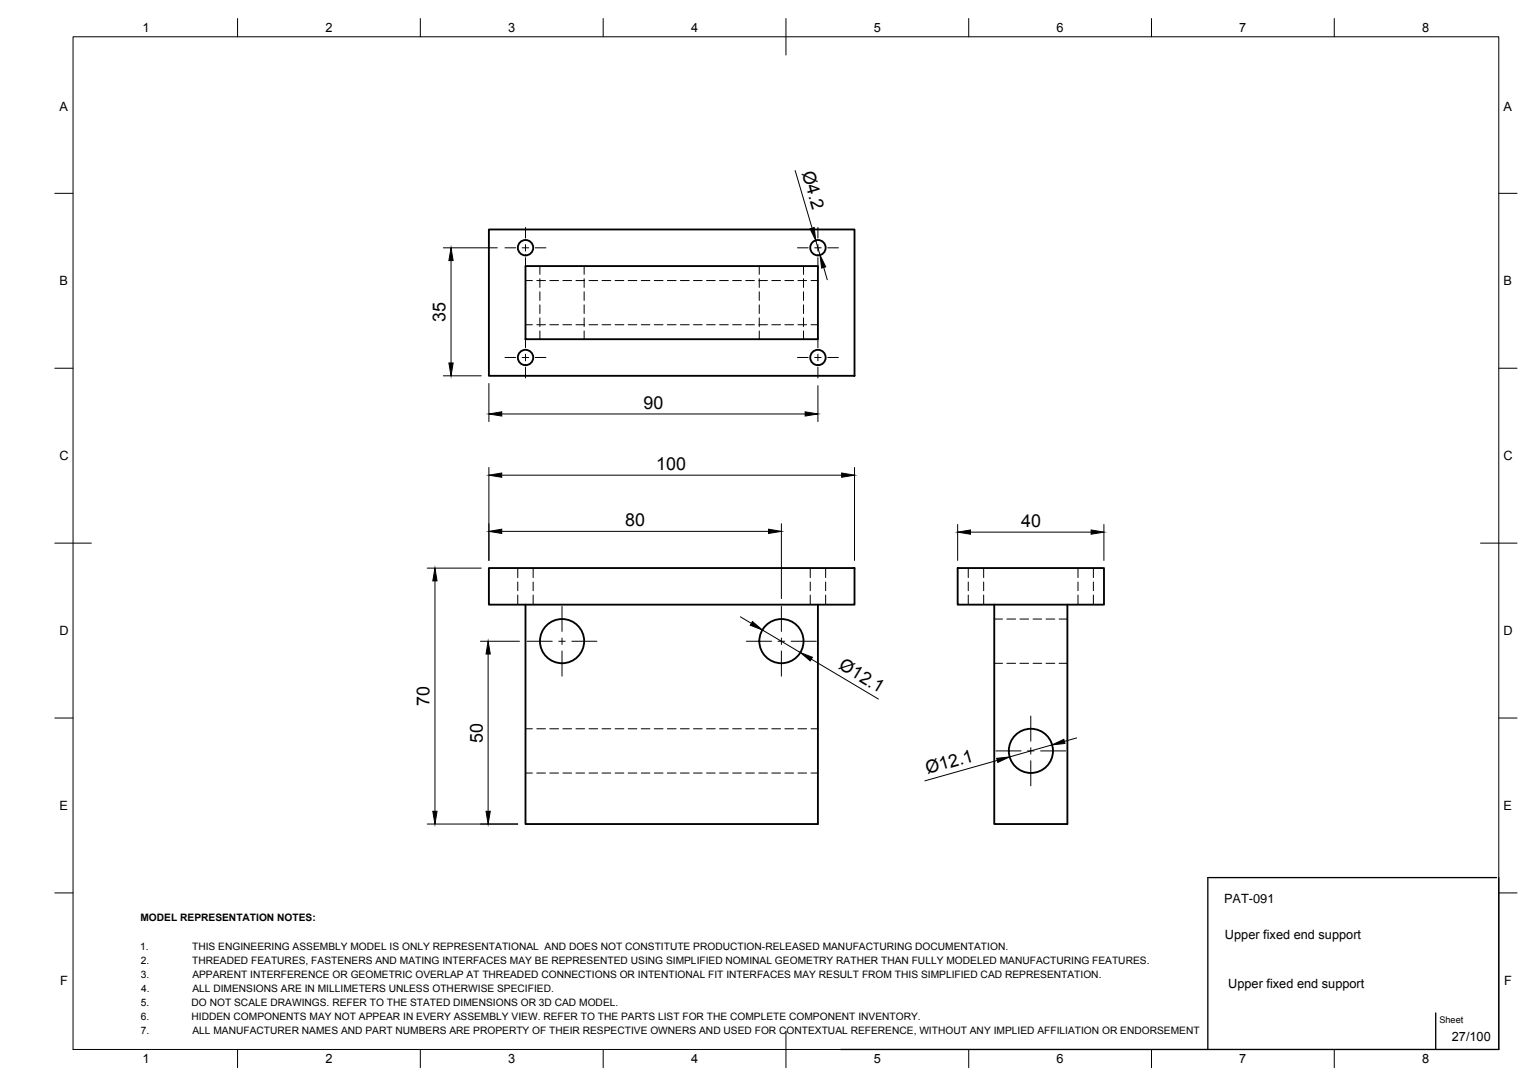
ISO-10303-21;
HEADER;
/* Generated by software containing ST-Developer
 * from STEP Tools, Inc. (www.steptools.com) 
 */

FILE_DESCRIPTION(
/* description */ ('PAT-091'),
/* implementation_level */ '2;1');

FILE_NAME(
/* name */ 'Upper fixed end support.step',
/* time_stamp */ '2026-10-27T15:34:44-07:00',
/* author */ (''),
/* organization */ (''),
/* preprocessor_version */ 'ST-DEVELOPER v20.2',
/* originating_system */ 'Autodesk Translation Framework v15.17.0.0',
/* authorisation */ '');

FILE_SCHEMA (('AUTOMOTIVE_DESIGN { 1 0 10303 214 3 1 1 }'));
ENDSEC;

DATA;
#10=MECHANICAL_DESIGN_GEOMETRIC_PRESENTATION_REPRESENTATION('',(#990),#25100);
#770=SHAPE_REPRESENTATION_RELATIONSHIP('SRR','None',#25532,#880);
#880=ADVANCED_BREP_SHAPE_REPRESENTATION('',(#1113),#25002);
#990=STYLED_ITEM('',(#26184),#1113);
#1113=MANIFOLD_SOLID_BREP('Body1',#13268);
#1350=FACE_BOUND('',#3193,.T.);
#1351=FACE_BOUND('',#3194,.T.);
#1352=FACE_BOUND('',#3195,.T.);
#1353=FACE_BOUND('',#3196,.T.);
#1354=FACE_BOUND('',#3197,.T.);
#1355=FACE_BOUND('',#3203,.T.);
#1356=FACE_BOUND('',#3205,.T.);
#1357=FACE_BOUND('',#3206,.T.);
#1358=FACE_BOUND('',#3211,.T.);
#1359=FACE_BOUND('',#3213,.T.);
#1360=FACE_BOUND('',#3214,.T.);
#1361=FACE_BOUND('',#3216,.T.);
#1362=FACE_BOUND('',#3217,.T.);
#1363=FACE_BOUND('',#3218,.T.);
#1364=FACE_BOUND('',#3219,.T.);
#1725=PLANE('',#14963);
#1726=PLANE('',#14964);
#1727=PLANE('',#14965);
#1728=PLANE('',#14966);
#1729=PLANE('',#14967);
#1730=PLANE('',#14968);
#1731=PLANE('',#14970);
#1732=PLANE('',#14979);
#1733=PLANE('',#14980);
#1734=PLANE('',#14981);
#1735=PLANE('',#14982);
#2235=FACE_OUTER_BOUND('',#3188,.T.);
#2236=FACE_OUTER_BOUND('',#3189,.T.);
#2237=FACE_OUTER_BOUND('',#3190,.T.);
#2238=FACE_OUTER_BOUND('',#3191,.T.);
#2239=FACE_OUTER_BOUND('',#3192,.T.);
#2240=FACE_OUTER_BOUND('',#3198,.T.);
#2241=FACE_OUTER_BOUND('',#3199,.T.);
#2242=FACE_OUTER_BOUND('',#3200,.T.);
#2243=FACE_OUTER_BOUND('',#3201,.T.);
#2244=FACE_OUTER_BOUND('',#3202,.T.);
#2245=FACE_OUTER_BOUND('',#3204,.T.);
#2246=FACE_OUTER_BOUND('',#3207,.T.);
#2247=FACE_OUTER_BOUND('',#3208,.T.);
#2248=FACE_OUTER_BOUND('',#3209,.T.);
#2249=FACE_OUTER_BOUND('',#3210,.T.);
#2250=FACE_OUTER_BOUND('',#3212,.T.);
#2251=FACE_OUTER_BOUND('',#3215,.T.);
#2252=FACE_OUTER_BOUND('',#3220,.T.);
#3188=EDGE_LOOP('',(#9716,#9717,#9718,#9719));
#3189=EDGE_LOOP('',(#9720,#9721,#9722,#9723));
#3190=EDGE_LOOP('',(#9724,#9725,#9726,#9727));
#3191=EDGE_LOOP('',(#9728,#9729,#9730,#9731));
#3192=EDGE_LOOP('',(#9732,#9733,#9734,#9735));
#3193=EDGE_LOOP('',(#9736,#9737,#9738,#9739));
#3194=EDGE_LOOP('',(#9740));
#3195=EDGE_LOOP('',(#9741));
#3196=EDGE_LOOP('',(#9742));
#3197=EDGE_LOOP('',(#9743));
#3198=EDGE_LOOP('',(#9744,#9745,#9746,#9747));
#3199=EDGE_LOOP('',(#9748,#9749,#9750,#9751));
#3200=EDGE_LOOP('',(#9752,#9753,#9754,#9755));
#3201=EDGE_LOOP('',(#9756,#9757,#9758,#9759));
#3202=EDGE_LOOP('',(#9760,#9761,#9762,#9763));
#3203=EDGE_LOOP('',(#9764));
#3204=EDGE_LOOP('',(#9765,#9766,#9767,#9768));
#3205=EDGE_LOOP('',(#9769));
#3206=EDGE_LOOP('',(#9770));
#3207=EDGE_LOOP('',(#9771,#9772,#9773,#9774));
#3208=EDGE_LOOP('',(#9775,#9776,#9777,#9778));
#3209=EDGE_LOOP('',(#9779,#9780,#9781,#9782));
#3210=EDGE_LOOP('',(#9783,#9784,#9785,#9786));
#3211=EDGE_LOOP('',(#9787));
#3212=EDGE_LOOP('',(#9788,#9789,#9790,#9791));
#3213=EDGE_LOOP('',(#9792));
#3214=EDGE_LOOP('',(#9793));
#3215=EDGE_LOOP('',(#9794,#9795,#9796,#9797));
#3216=EDGE_LOOP('',(#9798));
#3217=EDGE_LOOP('',(#9799));
#3218=EDGE_LOOP('',(#9800));
#3219=EDGE_LOOP('',(#9801));
#3220=EDGE_LOOP('',(#9802,#9803,#9804,#9805));
#4325=LINE('',#21792,#5065);
#4326=LINE('',#21798,#5066);
#4327=LINE('',#21804,#5067);
#4328=LINE('',#21810,#5068);
#4329=LINE('',#21815,#5069);
#4330=LINE('',#21817,#5070);
#4331=LINE('',#21819,#5071);
#4332=LINE('',#21820,#5072);
#4333=LINE('',#21823,#5073);
#4334=LINE('',#21825,#5074);
#4335=LINE('',#21827,#5075);
#4336=LINE('',#21828,#5076);
#4337=LINE('',#21831,#5077);
#4338=LINE('',#21833,#5078);
#4339=LINE('',#21834,#5079);
#4340=LINE('',#21837,#5080);
#4341=LINE('',#21838,#5081);
#4342=LINE('',#21841,#5082);
#4343=LINE('',#21842,#5083);
#4344=LINE('',#21844,#5084);
#4345=LINE('',#21847,#5085);
#4346=LINE('',#21849,#5086);
#4347=LINE('',#21850,#5087);
#4348=LINE('',#21855,#5088);
#4349=LINE('',#21856,#5089);
#4350=LINE('',#21863,#5090);
#4351=LINE('',#21867,#5091);
#4352=LINE('',#21871,#5092);
#4353=LINE('',#21875,#5093);
#4354=LINE('',#21876,#5094);
#4355=LINE('',#21878,#5095);
#5065=VECTOR('',#17405,0.21);
#5066=VECTOR('',#17412,0.21);
#5067=VECTOR('',#17419,0.21);
#5068=VECTOR('',#17426,0.21);
#5069=VECTOR('',#17431,1.);
#5070=VECTOR('',#17432,1.);
#5071=VECTOR('',#17433,1.);
#5072=VECTOR('',#17434,1.);
#5073=VECTOR('',#17435,1.);
#5074=VECTOR('',#17436,1.);
#5075=VECTOR('',#17437,1.);
#5076=VECTOR('',#17438,1.);
#5077=VECTOR('',#17441,1.);
#5078=VECTOR('',#17442,1.);
#5079=VECTOR('',#17443,1.);
#5080=VECTOR('',#17446,1.);
#5081=VECTOR('',#17447,1.);
#5082=VECTOR('',#17450,1.);
#5083=VECTOR('',#17451,1.);
#5084=VECTOR('',#17454,1.);
#5085=VECTOR('',#17457,1.);
#5086=VECTOR('',#17458,1.);
#5087=VECTOR('',#17459,1.);
#5088=VECTOR('',#17464,1.);
#5089=VECTOR('',#17465,1.);
#5090=VECTOR('',#17472,0.605);
#5091=VECTOR('',#17477,0.605);
#5092=VECTOR('',#17482,0.605);
#5093=VECTOR('',#17487,1.);
#5094=VECTOR('',#17488,1.);
#5095=VECTOR('',#17491,1.);
#5775=CIRCLE('',#14952,0.21);
#5776=CIRCLE('',#14953,0.21);
#5777=CIRCLE('',#14955,0.21);
#5778=CIRCLE('',#14956,0.21);
#5779=CIRCLE('',#14958,0.21);
#5780=CIRCLE('',#14959,0.21);
#5781=CIRCLE('',#14961,0.21);
#5782=CIRCLE('',#14962,0.21);
#5783=CIRCLE('',#14969,0.605);
#5784=CIRCLE('',#14971,0.605);
#5785=CIRCLE('',#14972,0.605);
#5786=CIRCLE('',#14974,0.605);
#5787=CIRCLE('',#14976,0.605);
#5788=CIRCLE('',#14978,0.605);
#6630=VERTEX_POINT('',#21789);
#6631=VERTEX_POINT('',#21791);
#6632=VERTEX_POINT('',#21795);
#6633=VERTEX_POINT('',#21797);
#6634=VERTEX_POINT('',#21801);
#6635=VERTEX_POINT('',#21803);
#6636=VERTEX_POINT('',#21807);
#6637=VERTEX_POINT('',#21809);
#6638=VERTEX_POINT('',#21813);
#6639=VERTEX_POINT('',#21814);
#6640=VERTEX_POINT('',#21816);
#6641=VERTEX_POINT('',#21818);
#6642=VERTEX_POINT('',#21821);
#6643=VERTEX_POINT('',#21822);
#6644=VERTEX_POINT('',#21824);
#6645=VERTEX_POINT('',#21826);
#6646=VERTEX_POINT('',#21830);
#6647=VERTEX_POINT('',#21832);
#6648=VERTEX_POINT('',#21836);
#6649=VERTEX_POINT('',#21840);
#6650=VERTEX_POINT('',#21846);
#6651=VERTEX_POINT('',#21848);
#6652=VERTEX_POINT('',#21851);
#6653=VERTEX_POINT('',#21854);
#6654=VERTEX_POINT('',#21857);
#6655=VERTEX_POINT('',#21859);
#6656=VERTEX_POINT('',#21862);
#6657=VERTEX_POINT('',#21866);
#6658=VERTEX_POINT('',#21870);
#6659=VERTEX_POINT('',#21874);
#7793=EDGE_CURVE('',#6630,#6630,#5775,.T.);
#7794=EDGE_CURVE('',#6630,#6631,#4325,.T.);
#7795=EDGE_CURVE('',#6631,#6631,#5776,.T.);
#7796=EDGE_CURVE('',#6632,#6632,#5777,.T.);
#7797=EDGE_CURVE('',#6632,#6633,#4326,.T.);
#7798=EDGE_CURVE('',#6633,#6633,#5778,.T.);
#7799=EDGE_CURVE('',#6634,#6634,#5779,.T.);
#7800=EDGE_CURVE('',#6634,#6635,#4327,.T.);
#7801=EDGE_CURVE('',#6635,#6635,#5780,.T.);
#7802=EDGE_CURVE('',#6636,#6636,#5781,.T.);
#7803=EDGE_CURVE('',#6636,#6637,#4328,.T.);
#7804=EDGE_CURVE('',#6637,#6637,#5782,.T.);
#7805=EDGE_CURVE('',#6638,#6639,#4329,.T.);
#7806=EDGE_CURVE('',#6640,#6638,#4330,.T.);
#7807=EDGE_CURVE('',#6641,#6640,#4331,.T.);
#7808=EDGE_CURVE('',#6639,#6641,#4332,.T.);
#7809=EDGE_CURVE('',#6642,#6643,#4333,.T.);
#7810=EDGE_CURVE('',#6644,#6642,#4334,.T.);
#7811=EDGE_CURVE('',#6645,#6644,#4335,.T.);
#7812=EDGE_CURVE('',#6643,#6645,#4336,.T.);
#7813=EDGE_CURVE('',#6638,#6646,#4337,.T.);
#7814=EDGE_CURVE('',#6647,#6646,#4338,.T.);
#7815=EDGE_CURVE('',#6640,#6647,#4339,.T.);
#7816=EDGE_CURVE('',#6648,#6647,#4340,.T.);
#7817=EDGE_CURVE('',#6641,#6648,#4341,.T.);
#7818=EDGE_CURVE('',#6649,#6648,#4342,.T.);
#7819=EDGE_CURVE('',#6639,#6649,#4343,.T.);
#7820=EDGE_CURVE('',#6646,#6649,#4344,.T.);
#7821=EDGE_CURVE('',#6650,#6644,#4345,.T.);
#7822=EDGE_CURVE('',#6650,#6651,#4346,.T.);
#7823=EDGE_CURVE('',#6651,#6645,#4347,.T.);
#7824=EDGE_CURVE('',#6652,#6652,#5783,.T.);
#7825=EDGE_CURVE('',#6653,#6642,#4348,.T.);
#7826=EDGE_CURVE('',#6653,#6650,#4349,.T.);
#7827=EDGE_CURVE('',#6654,#6654,#5784,.T.);
#7828=EDGE_CURVE('',#6655,#6655,#5785,.T.);
#7829=EDGE_CURVE('',#6652,#6656,#4350,.T.);
#7830=EDGE_CURVE('',#6656,#6656,#5786,.T.);
#7831=EDGE_CURVE('',#6655,#6657,#4351,.T.);
#7832=EDGE_CURVE('',#6657,#6657,#5787,.T.);
#7833=EDGE_CURVE('',#6654,#6658,#4352,.T.);
#7834=EDGE_CURVE('',#6658,#6658,#5788,.T.);
#7835=EDGE_CURVE('',#6659,#6643,#4353,.T.);
#7836=EDGE_CURVE('',#6659,#6653,#4354,.T.);
#7837=EDGE_CURVE('',#6651,#6659,#4355,.T.);
#9716=ORIENTED_EDGE('',*,*,#7793,.F.);
#9717=ORIENTED_EDGE('',*,*,#7794,.T.);
#9718=ORIENTED_EDGE('',*,*,#7795,.F.);
#9719=ORIENTED_EDGE('',*,*,#7794,.F.);
#9720=ORIENTED_EDGE('',*,*,#7796,.F.);
#9721=ORIENTED_EDGE('',*,*,#7797,.T.);
#9722=ORIENTED_EDGE('',*,*,#7798,.F.);
#9723=ORIENTED_EDGE('',*,*,#7797,.F.);
#9724=ORIENTED_EDGE('',*,*,#7799,.F.);
#9725=ORIENTED_EDGE('',*,*,#7800,.T.);
#9726=ORIENTED_EDGE('',*,*,#7801,.F.);
#9727=ORIENTED_EDGE('',*,*,#7800,.F.);
#9728=ORIENTED_EDGE('',*,*,#7802,.F.);
#9729=ORIENTED_EDGE('',*,*,#7803,.T.);
#9730=ORIENTED_EDGE('',*,*,#7804,.F.);
#9731=ORIENTED_EDGE('',*,*,#7803,.F.);
#9732=ORIENTED_EDGE('',*,*,#7805,.F.);
#9733=ORIENTED_EDGE('',*,*,#7806,.F.);
#9734=ORIENTED_EDGE('',*,*,#7807,.F.);
#9735=ORIENTED_EDGE('',*,*,#7808,.F.);
#9736=ORIENTED_EDGE('',*,*,#7809,.F.);
#9737=ORIENTED_EDGE('',*,*,#7810,.F.);
#9738=ORIENTED_EDGE('',*,*,#7811,.F.);
#9739=ORIENTED_EDGE('',*,*,#7812,.F.);
#9740=ORIENTED_EDGE('',*,*,#7802,.T.);
#9741=ORIENTED_EDGE('',*,*,#7799,.T.);
#9742=ORIENTED_EDGE('',*,*,#7796,.T.);
#9743=ORIENTED_EDGE('',*,*,#7793,.T.);
#9744=ORIENTED_EDGE('',*,*,#7806,.T.);
#9745=ORIENTED_EDGE('',*,*,#7813,.T.);
#9746=ORIENTED_EDGE('',*,*,#7814,.F.);
#9747=ORIENTED_EDGE('',*,*,#7815,.F.);
#9748=ORIENTED_EDGE('',*,*,#7807,.T.);
#9749=ORIENTED_EDGE('',*,*,#7815,.T.);
#9750=ORIENTED_EDGE('',*,*,#7816,.F.);
#9751=ORIENTED_EDGE('',*,*,#7817,.F.);
#9752=ORIENTED_EDGE('',*,*,#7808,.T.);
#9753=ORIENTED_EDGE('',*,*,#7817,.T.);
#9754=ORIENTED_EDGE('',*,*,#7818,.F.);
#9755=ORIENTED_EDGE('',*,*,#7819,.F.);
#9756=ORIENTED_EDGE('',*,*,#7805,.T.);
#9757=ORIENTED_EDGE('',*,*,#7819,.T.);
#9758=ORIENTED_EDGE('',*,*,#7820,.F.);
#9759=ORIENTED_EDGE('',*,*,#7813,.F.);
#9760=ORIENTED_EDGE('',*,*,#7811,.T.);
#9761=ORIENTED_EDGE('',*,*,#7821,.F.);
#9762=ORIENTED_EDGE('',*,*,#7822,.T.);
#9763=ORIENTED_EDGE('',*,*,#7823,.T.);
#9764=ORIENTED_EDGE('',*,*,#7824,.T.);
#9765=ORIENTED_EDGE('',*,*,#7810,.T.);
#9766=ORIENTED_EDGE('',*,*,#7825,.F.);
#9767=ORIENTED_EDGE('',*,*,#7826,.T.);
#9768=ORIENTED_EDGE('',*,*,#7821,.T.);
#9769=ORIENTED_EDGE('',*,*,#7827,.T.);
#9770=ORIENTED_EDGE('',*,*,#7828,.T.);
#9771=ORIENTED_EDGE('',*,*,#7824,.F.);
#9772=ORIENTED_EDGE('',*,*,#7829,.T.);
#9773=ORIENTED_EDGE('',*,*,#7830,.F.);
#9774=ORIENTED_EDGE('',*,*,#7829,.F.);
#9775=ORIENTED_EDGE('',*,*,#7828,.F.);
#9776=ORIENTED_EDGE('',*,*,#7831,.T.);
#9777=ORIENTED_EDGE('',*,*,#7832,.F.);
#9778=ORIENTED_EDGE('',*,*,#7831,.F.);
#9779=ORIENTED_EDGE('',*,*,#7827,.F.);
#9780=ORIENTED_EDGE('',*,*,#7833,.T.);
#9781=ORIENTED_EDGE('',*,*,#7834,.F.);
#9782=ORIENTED_EDGE('',*,*,#7833,.F.);
#9783=ORIENTED_EDGE('',*,*,#7809,.T.);
#9784=ORIENTED_EDGE('',*,*,#7835,.F.);
#9785=ORIENTED_EDGE('',*,*,#7836,.T.);
#9786=ORIENTED_EDGE('',*,*,#7825,.T.);
#9787=ORIENTED_EDGE('',*,*,#7830,.T.);
#9788=ORIENTED_EDGE('',*,*,#7812,.T.);
#9789=ORIENTED_EDGE('',*,*,#7823,.F.);
#9790=ORIENTED_EDGE('',*,*,#7837,.T.);
#9791=ORIENTED_EDGE('',*,*,#7835,.T.);
#9792=ORIENTED_EDGE('',*,*,#7832,.T.);
#9793=ORIENTED_EDGE('',*,*,#7834,.T.);
#9794=ORIENTED_EDGE('',*,*,#7820,.T.);
#9795=ORIENTED_EDGE('',*,*,#7818,.T.);
#9796=ORIENTED_EDGE('',*,*,#7816,.T.);
#9797=ORIENTED_EDGE('',*,*,#7814,.T.);
#9798=ORIENTED_EDGE('',*,*,#7795,.T.);
#9799=ORIENTED_EDGE('',*,*,#7798,.T.);
#9800=ORIENTED_EDGE('',*,*,#7801,.T.);
#9801=ORIENTED_EDGE('',*,*,#7804,.T.);
#9802=ORIENTED_EDGE('',*,*,#7826,.F.);
#9803=ORIENTED_EDGE('',*,*,#7836,.F.);
#9804=ORIENTED_EDGE('',*,*,#7837,.F.);
#9805=ORIENTED_EDGE('',*,*,#7822,.F.);
#12158=CYLINDRICAL_SURFACE('',#14951,0.21);
#12159=CYLINDRICAL_SURFACE('',#14954,0.21);
#12160=CYLINDRICAL_SURFACE('',#14957,0.21);
#12161=CYLINDRICAL_SURFACE('',#14960,0.21);
#12162=CYLINDRICAL_SURFACE('',#14973,0.605);
#12163=CYLINDRICAL_SURFACE('',#14975,0.605);
#12164=CYLINDRICAL_SURFACE('',#14977,0.605);
#12602=ADVANCED_FACE('',(#2235),#12158,.F.);
#12603=ADVANCED_FACE('',(#2236),#12159,.F.);
#12604=ADVANCED_FACE('',(#2237),#12160,.F.);
#12605=ADVANCED_FACE('',(#2238),#12161,.F.);
#12606=ADVANCED_FACE('',(#2239,#1350,#1351,#1352,#1353,#1354),#1725,.F.);
#12607=ADVANCED_FACE('',(#2240),#1726,.T.);
#12608=ADVANCED_FACE('',(#2241),#1727,.T.);
#12609=ADVANCED_FACE('',(#2242),#1728,.T.);
#12610=ADVANCED_FACE('',(#2243),#1729,.T.);
#12611=ADVANCED_FACE('',(#2244,#1355),#1730,.T.);
#12612=ADVANCED_FACE('',(#2245,#1356,#1357),#1731,.T.);
#12613=ADVANCED_FACE('',(#2246),#12162,.F.);
#12614=ADVANCED_FACE('',(#2247),#12163,.F.);
#12615=ADVANCED_FACE('',(#2248),#12164,.F.);
#12616=ADVANCED_FACE('',(#2249,#1358),#1732,.T.);
#12617=ADVANCED_FACE('',(#2250,#1359,#1360),#1733,.T.);
#12618=ADVANCED_FACE('',(#2251,#1361,#1362,#1363,#1364),#1734,.T.);
#12619=ADVANCED_FACE('',(#2252),#1735,.F.);
#13268=CLOSED_SHELL('',(#12602,#12603,#12604,#12605,#12606,#12607,#12608,
#12609,#12610,#12611,#12612,#12613,#12614,#12615,#12616,#12617,#12618,#12619));
#14950=AXIS2_PLACEMENT_3D('',#21787,#17399,#17400);
#14951=AXIS2_PLACEMENT_3D('',#21788,#17401,#17402);
#14952=AXIS2_PLACEMENT_3D('',#21790,#17403,#17404);
#14953=AXIS2_PLACEMENT_3D('',#21793,#17406,#17407);
#14954=AXIS2_PLACEMENT_3D('',#21794,#17408,#17409);
#14955=AXIS2_PLACEMENT_3D('',#21796,#17410,#17411);
#14956=AXIS2_PLACEMENT_3D('',#21799,#17413,#17414);
#14957=AXIS2_PLACEMENT_3D('',#21800,#17415,#17416);
#14958=AXIS2_PLACEMENT_3D('',#21802,#17417,#17418);
#14959=AXIS2_PLACEMENT_3D('',#21805,#17420,#17421);
#14960=AXIS2_PLACEMENT_3D('',#21806,#17422,#17423);
#14961=AXIS2_PLACEMENT_3D('',#21808,#17424,#17425);
#14962=AXIS2_PLACEMENT_3D('',#21811,#17427,#17428);
#14963=AXIS2_PLACEMENT_3D('',#21812,#17429,#17430);
#14964=AXIS2_PLACEMENT_3D('',#21829,#17439,#17440);
#14965=AXIS2_PLACEMENT_3D('',#21835,#17444,#17445);
#14966=AXIS2_PLACEMENT_3D('',#21839,#17448,#17449);
#14967=AXIS2_PLACEMENT_3D('',#21843,#17452,#17453);
#14968=AXIS2_PLACEMENT_3D('',#21845,#17455,#17456);
#14969=AXIS2_PLACEMENT_3D('',#21852,#17460,#17461);
#14970=AXIS2_PLACEMENT_3D('',#21853,#17462,#17463);
#14971=AXIS2_PLACEMENT_3D('',#21858,#17466,#17467);
#14972=AXIS2_PLACEMENT_3D('',#21860,#17468,#17469);
#14973=AXIS2_PLACEMENT_3D('',#21861,#17470,#17471);
#14974=AXIS2_PLACEMENT_3D('',#21864,#17473,#17474);
#14975=AXIS2_PLACEMENT_3D('',#21865,#17475,#17476);
#14976=AXIS2_PLACEMENT_3D('',#21868,#17478,#17479);
#14977=AXIS2_PLACEMENT_3D('',#21869,#17480,#17481);
#14978=AXIS2_PLACEMENT_3D('',#21872,#17483,#17484);
#14979=AXIS2_PLACEMENT_3D('',#21873,#17485,#17486);
#14980=AXIS2_PLACEMENT_3D('',#21877,#17489,#17490);
#14981=AXIS2_PLACEMENT_3D('',#21879,#17492,#17493);
#14982=AXIS2_PLACEMENT_3D('',#21880,#17494,#17495);
#17399=DIRECTION('axis',(0.,0.,1.));
#17400=DIRECTION('refdir',(1.,0.,0.));
#17401=DIRECTION('center_axis',(0.,0.,1.));
#17402=DIRECTION('ref_axis',(1.,0.,0.));
#17403=DIRECTION('center_axis',(0.,0.,1.));
#17404=DIRECTION('ref_axis',(1.,0.,0.));
#17405=DIRECTION('',(0.,0.,1.));
#17406=DIRECTION('center_axis',(0.,0.,-1.));
#17407=DIRECTION('ref_axis',(1.,0.,0.));
#17408=DIRECTION('center_axis',(0.,0.,1.));
#17409=DIRECTION('ref_axis',(1.,0.,0.));
#17410=DIRECTION('center_axis',(0.,0.,1.));
#17411=DIRECTION('ref_axis',(1.,0.,0.));
#17412=DIRECTION('',(0.,0.,1.));
#17413=DIRECTION('center_axis',(0.,0.,-1.));
#17414=DIRECTION('ref_axis',(1.,0.,0.));
#17415=DIRECTION('center_axis',(0.,0.,1.));
#17416=DIRECTION('ref_axis',(1.,0.,0.));
#17417=DIRECTION('center_axis',(0.,0.,1.));
#17418=DIRECTION('ref_axis',(1.,0.,0.));
#17419=DIRECTION('',(0.,0.,1.));
#17420=DIRECTION('center_axis',(0.,0.,-1.));
#17421=DIRECTION('ref_axis',(1.,0.,0.));
#17422=DIRECTION('center_axis',(0.,0.,1.));
#17423=DIRECTION('ref_axis',(1.,0.,0.));
#17424=DIRECTION('center_axis',(0.,0.,1.));
#17425=DIRECTION('ref_axis',(1.,0.,0.));
#17426=DIRECTION('',(0.,0.,1.));
#17427=DIRECTION('center_axis',(0.,0.,-1.));
#17428=DIRECTION('ref_axis',(1.,0.,0.));
#17429=DIRECTION('center_axis',(0.,0.,1.));
#17430=DIRECTION('ref_axis',(1.,0.,0.));
#17431=DIRECTION('',(0.,-1.,0.));
#17432=DIRECTION('',(-1.,0.,0.));
#17433=DIRECTION('',(0.,1.,0.));
#17434=DIRECTION('',(1.,0.,0.));
#17435=DIRECTION('',(1.,0.,0.));
#17436=DIRECTION('',(0.,1.,0.));
#17437=DIRECTION('',(-1.,0.,0.));
#17438=DIRECTION('',(0.,-1.,0.));
#17439=DIRECTION('center_axis',(0.,1.,0.));
#17440=DIRECTION('ref_axis',(-1.,0.,0.));
#17441=DIRECTION('',(0.,0.,1.));
#17442=DIRECTION('',(-1.,0.,0.));
#17443=DIRECTION('',(0.,0.,1.));
#17444=DIRECTION('center_axis',(1.,0.,0.));
#17445=DIRECTION('ref_axis',(0.,1.,0.));
#17446=DIRECTION('',(0.,1.,0.));
#17447=DIRECTION('',(0.,0.,1.));
#17448=DIRECTION('center_axis',(0.,-1.,0.));
#17449=DIRECTION('ref_axis',(1.,0.,0.));
#17450=DIRECTION('',(1.,0.,0.));
#17451=DIRECTION('',(0.,0.,1.));
#17452=DIRECTION('center_axis',(-1.,0.,0.));
#17453=DIRECTION('ref_axis',(0.,-1.,0.));
#17454=DIRECTION('',(0.,-1.,0.));
#17455=DIRECTION('center_axis',(0.,-1.,0.));
#17456=DIRECTION('ref_axis',(1.,0.,0.));
#17457=DIRECTION('',(0.,0.,1.));
#17458=DIRECTION('',(1.,0.,0.));
#17459=DIRECTION('',(0.,0.,1.));
#17460=DIRECTION('center_axis',(0.,1.,0.));
#17461=DIRECTION('ref_axis',(1.,0.,0.));
#17462=DIRECTION('center_axis',(-1.,0.,0.));
#17463=DIRECTION('ref_axis',(0.,-1.,0.));
#17464=DIRECTION('',(0.,0.,1.));
#17465=DIRECTION('',(0.,-1.,0.));
#17466=DIRECTION('center_axis',(1.,0.,0.));
#17467=DIRECTION('ref_axis',(0.,0.,-1.));
#17468=DIRECTION('center_axis',(1.,0.,0.));
#17469=DIRECTION('ref_axis',(0.,0.,-1.));
#17470=DIRECTION('center_axis',(0.,1.,0.));
#17471=DIRECTION('ref_axis',(1.,0.,0.));
#17472=DIRECTION('',(0.,1.,0.));
#17473=DIRECTION('center_axis',(0.,-1.,0.));
#17474=DIRECTION('ref_axis',(1.,0.,0.));
#17475=DIRECTION('center_axis',(1.,0.,0.));
#17476=DIRECTION('ref_axis',(0.,0.,-1.));
#17477=DIRECTION('',(1.,0.,0.));
#17478=DIRECTION('center_axis',(-1.,0.,0.));
#17479=DIRECTION('ref_axis',(0.,0.,-1.));
#17480=DIRECTION('center_axis',(1.,0.,0.));
#17481=DIRECTION('ref_axis',(0.,0.,-1.));
#17482=DIRECTION('',(1.,0.,0.));
#17483=DIRECTION('center_axis',(-1.,0.,0.));
#17484=DIRECTION('ref_axis',(0.,0.,-1.));
#17485=DIRECTION('center_axis',(0.,1.,0.));
#17486=DIRECTION('ref_axis',(-1.,0.,0.));
#17487=DIRECTION('',(0.,0.,1.));
#17488=DIRECTION('',(-1.,0.,0.));
#17489=DIRECTION('center_axis',(1.,0.,0.));
#17490=DIRECTION('ref_axis',(0.,1.,0.));
#17491=DIRECTION('',(0.,1.,0.));
#17492=DIRECTION('center_axis',(0.,0.,1.));
#17493=DIRECTION('ref_axis',(1.,0.,0.));
#17494=DIRECTION('center_axis',(0.,0.,1.));
#17495=DIRECTION('ref_axis',(1.,0.,0.));
#21787=CARTESIAN_POINT('',(0.,0.,0.));
#21788=CARTESIAN_POINT('Origin',(1.5,-4.,16.9));
#21789=CARTESIAN_POINT('',(1.29,-4.,17.));
#21790=CARTESIAN_POINT('Origin',(1.5,-4.,17.));
#21791=CARTESIAN_POINT('',(1.29,-4.,18.));
#21792=CARTESIAN_POINT('',(1.29,-4.,16.9));
#21793=CARTESIAN_POINT('Origin',(1.5,-4.,18.));
#21794=CARTESIAN_POINT('Origin',(-1.5,4.,16.9));
#21795=CARTESIAN_POINT('',(-1.71,4.,17.));
#21796=CARTESIAN_POINT('Origin',(-1.5,4.,17.));
#21797=CARTESIAN_POINT('',(-1.71,4.,18.));
#21798=CARTESIAN_POINT('',(-1.71,4.,16.9));
#21799=CARTESIAN_POINT('Origin',(-1.5,4.,18.));
#21800=CARTESIAN_POINT('Origin',(-1.5,-4.,16.9));
#21801=CARTESIAN_POINT('',(-1.71,-4.,17.));
#21802=CARTESIAN_POINT('Origin',(-1.5,-4.,17.));
#21803=CARTESIAN_POINT('',(-1.71,-4.,18.));
#21804=CARTESIAN_POINT('',(-1.71,-4.,16.9));
#21805=CARTESIAN_POINT('Origin',(-1.5,-4.,18.));
#21806=CARTESIAN_POINT('Origin',(1.5,4.,16.9));
#21807=CARTESIAN_POINT('',(1.29,4.,17.));
#21808=CARTESIAN_POINT('Origin',(1.5,4.,17.));
#21809=CARTESIAN_POINT('',(1.29,4.,18.));
#21810=CARTESIAN_POINT('',(1.29,4.,16.9));
#21811=CARTESIAN_POINT('Origin',(1.5,4.,18.));
#21812=CARTESIAN_POINT('Origin',(0.,0.,17.));
#21813=CARTESIAN_POINT('',(-2.,5.,17.));
#21814=CARTESIAN_POINT('',(-2.,-5.,17.));
#21815=CARTESIAN_POINT('',(-2.,5.,17.));
#21816=CARTESIAN_POINT('',(2.,5.,17.));
#21817=CARTESIAN_POINT('',(2.,5.,17.));
#21818=CARTESIAN_POINT('',(2.,-5.,17.));
#21819=CARTESIAN_POINT('',(2.,-5.,17.));
#21820=CARTESIAN_POINT('',(-2.,-5.,17.));
#21821=CARTESIAN_POINT('',(-1.,4.,17.));
#21822=CARTESIAN_POINT('',(1.,4.,17.));
#21823=CARTESIAN_POINT('',(0.5,4.,17.));
#21824=CARTESIAN_POINT('',(-1.,-4.,17.));
#21825=CARTESIAN_POINT('',(-1.,2.,17.));
#21826=CARTESIAN_POINT('',(1.,-4.,17.));
#21827=CARTESIAN_POINT('',(-0.5,-4.,17.));
#21828=CARTESIAN_POINT('',(1.,-2.,17.));
#21829=CARTESIAN_POINT('Origin',(2.,5.,17.));
#21830=CARTESIAN_POINT('',(-2.,5.,18.));
#21831=CARTESIAN_POINT('',(-2.,5.,17.));
#21832=CARTESIAN_POINT('',(2.,5.,18.));
#21833=CARTESIAN_POINT('',(2.,5.,18.));
#21834=CARTESIAN_POINT('',(2.,5.,17.));
#21835=CARTESIAN_POINT('Origin',(2.,-5.,17.));
#21836=CARTESIAN_POINT('',(2.,-5.,18.));
#21837=CARTESIAN_POINT('',(2.,-5.,18.));
#21838=CARTESIAN_POINT('',(2.,-5.,17.));
#21839=CARTESIAN_POINT('Origin',(-2.,-5.,17.));
#21840=CARTESIAN_POINT('',(-2.,-5.,18.));
#21841=CARTESIAN_POINT('',(-2.,-5.,18.));
#21842=CARTESIAN_POINT('',(-2.,-5.,17.));
#21843=CARTESIAN_POINT('Origin',(-2.,5.,17.));
#21844=CARTESIAN_POINT('',(-2.,5.,18.));
#21845=CARTESIAN_POINT('Origin',(-1.,-4.,11.));
#21846=CARTESIAN_POINT('',(-1.,-4.,11.));
#21847=CARTESIAN_POINT('',(-1.,-4.,11.));
#21848=CARTESIAN_POINT('',(1.,-4.,11.));
#21849=CARTESIAN_POINT('',(-1.,-4.,11.));
#21850=CARTESIAN_POINT('',(1.,-4.,11.));
#21851=CARTESIAN_POINT('',(-0.605,-4.,13.));
#21852=CARTESIAN_POINT('Origin',(0.,-4.,13.));
#21853=CARTESIAN_POINT('Origin',(-1.,4.,11.));
#21854=CARTESIAN_POINT('',(-1.,4.,11.));
#21855=CARTESIAN_POINT('',(-1.,4.,11.));
#21856=CARTESIAN_POINT('',(-1.,4.,11.));
#21857=CARTESIAN_POINT('',(-1.,3.,16.605));
#21858=CARTESIAN_POINT('Origin',(-1.,3.,16.));
#21859=CARTESIAN_POINT('',(-1.,-3.,16.605));
#21860=CARTESIAN_POINT('Origin',(-1.,-3.,16.));
#21861=CARTESIAN_POINT('Origin',(0.,-5.1,13.));
#21862=CARTESIAN_POINT('',(-0.605,4.,13.));
#21863=CARTESIAN_POINT('',(-0.605,-5.1,13.));
#21864=CARTESIAN_POINT('Origin',(0.,4.,13.));
#21865=CARTESIAN_POINT('Origin',(-1.1,-3.,16.));
#21866=CARTESIAN_POINT('',(1.,-3.,16.605));
#21867=CARTESIAN_POINT('',(-1.1,-3.,16.605));
#21868=CARTESIAN_POINT('Origin',(1.,-3.,16.));
#21869=CARTESIAN_POINT('Origin',(-1.1,3.,16.));
#21870=CARTESIAN_POINT('',(1.,3.,16.605));
#21871=CARTESIAN_POINT('',(-1.1,3.,16.605));
#21872=CARTESIAN_POINT('Origin',(1.,3.,16.));
#21873=CARTESIAN_POINT('Origin',(1.,4.,11.));
#21874=CARTESIAN_POINT('',(1.,4.,11.));
#21875=CARTESIAN_POINT('',(1.,4.,11.));
#21876=CARTESIAN_POINT('',(1.,4.,11.));
#21877=CARTESIAN_POINT('Origin',(1.,-4.,11.));
#21878=CARTESIAN_POINT('',(1.,-4.,11.));
#21879=CARTESIAN_POINT('Origin',(0.,0.,18.));
#21880=CARTESIAN_POINT('Origin',(0.,0.,11.));
#24881=UNCERTAINTY_MEASURE_WITH_UNIT(LENGTH_MEASURE(0.001),#25101,
'DISTANCE_ACCURACY_VALUE',
'Maximum model space distance between geometric entities at asserted c
onnectivities');
#24979=UNCERTAINTY_MEASURE_WITH_UNIT(LENGTH_MEASURE(0.001),#25101,
'DISTANCE_ACCURACY_VALUE',
'Maximum model space distance between geometric entities at asserted c
onnectivities');
#25002=(
GEOMETRIC_REPRESENTATION_CONTEXT(3)
GLOBAL_UNCERTAINTY_ASSIGNED_CONTEXT((#24881))
GLOBAL_UNIT_ASSIGNED_CONTEXT((#25101,#25103,#25104))
REPRESENTATION_CONTEXT('','3D')
);
#25100=(
GEOMETRIC_REPRESENTATION_CONTEXT(3)
GLOBAL_UNCERTAINTY_ASSIGNED_CONTEXT((#24979))
GLOBAL_UNIT_ASSIGNED_CONTEXT((#25101,#25103,#25104))
REPRESENTATION_CONTEXT('','3D')
);
#25101=(
LENGTH_UNIT()
NAMED_UNIT(*)
SI_UNIT(.CENTI.,.METRE.)
);
#25103=(
NAMED_UNIT(*)
PLANE_ANGLE_UNIT()
SI_UNIT($,.RADIAN.)
);
#25104=(
NAMED_UNIT(*)
SI_UNIT($,.STERADIAN.)
SOLID_ANGLE_UNIT()
);
#25127=SHAPE_DEFINITION_REPRESENTATION(#25247,#25532);
#25247=PRODUCT_DEFINITION_SHAPE('',$,#25653);
#25532=SHAPE_REPRESENTATION('',(#14950),#25002);
#25630=PRODUCT_DEFINITION_CONTEXT('part definition',#25992,'design');
#25653=PRODUCT_DEFINITION('Upper fixed end support',
'Upper fixed end support',#25773,#25630);
#25773=PRODUCT_DEFINITION_FORMATION('',$,#26016);
#25992=APPLICATION_CONTEXT(
'Core Data for Automotive Mechanical Design Process');
#25993=PRODUCT_CONTEXT('part definition',#25992,'mechanical');
#26016=PRODUCT('Upper fixed end support','Upper fixed end support',
'Upper fixed end support',(#25993));
#26178=COLOUR_RGB('Sky Blue',0.24,0.69,0.87);
#26179=FILL_AREA_STYLE_COLOUR('',#26178);
#26180=FILL_AREA_STYLE('',(#26179));
#26181=SURFACE_STYLE_FILL_AREA(#26180);
#26182=SURFACE_SIDE_STYLE('',(#26181));
#26183=SURFACE_STYLE_USAGE(.BOTH.,#26182);
#26184=PRESENTATION_STYLE_ASSIGNMENT((#26183));
ENDSEC;
END-ISO-10303-21;
